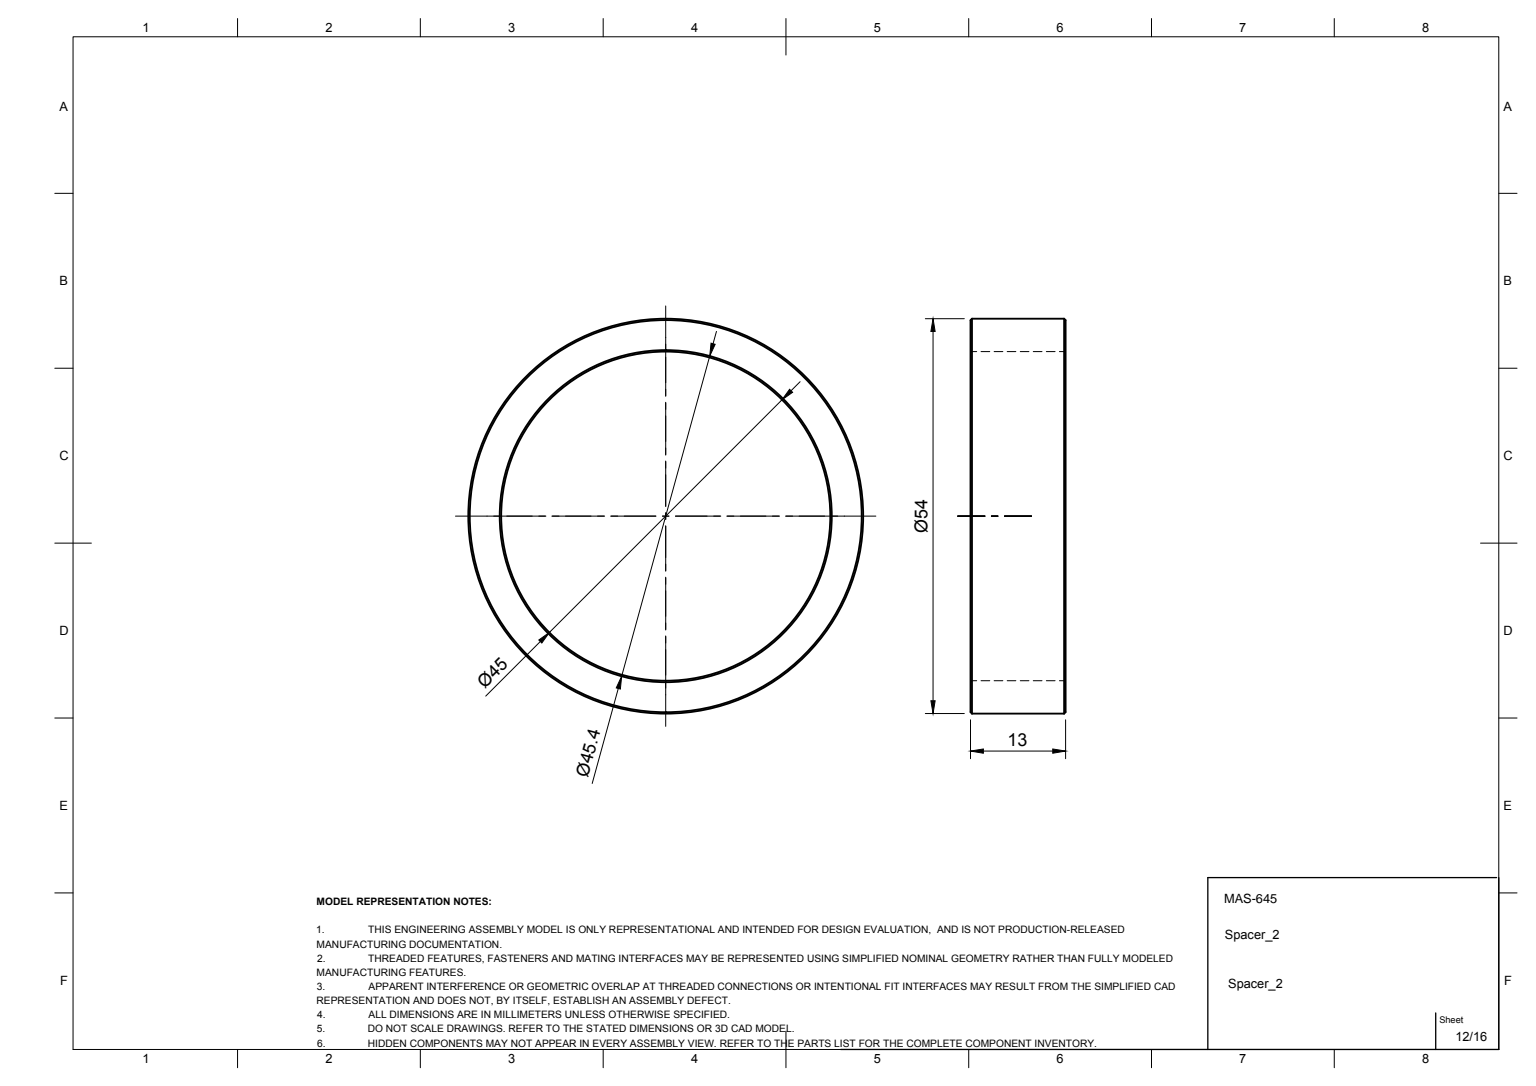
ISO-10303-21;
HEADER;
FILE_DESCRIPTION((''),'2;1');
FILE_NAME('Spacer_2.step','2026-10-09T10:54:55-07:00',(''),(''),'','','');
FILE_SCHEMA (('AUTOMOTIVE_DESIGN { 1 0 10303 214 3 1 1 }'));
ENDSEC;
DATA;
#10=MECHANICAL_DESIGN_GEOMETRIC_PRESENTATION_REPRESENTATION('',(#602),#63824);
#572=SHAPE_REPRESENTATION_RELATIONSHIP('SRR','None',#63886,#587) ;
#587=ADVANCED_BREP_SHAPE_REPRESENTATION('',(#617),#63816) ;
#602=STYLED_ITEM('',(#63963),#617) ;
#617=MANIFOLD_SOLID_BREP('Body1',#15501) ;
#748=FACE_BOUND('',#2811,.T.) ;
#749=FACE_BOUND('',#2817,.T.) ;
#906=PLANE('',#16195) ;
#907=PLANE('',#16205) ;
#1262=CYLINDRICAL_SURFACE('',#16197,27.) ;
#1263=CYLINDRICAL_SURFACE('',#16201,22.5) ;
#1825=FACE_OUTER_BOUND('',#2809,.T.) ;
#1826=FACE_OUTER_BOUND('',#2810,.T.) ;
#1827=FACE_OUTER_BOUND('',#2812,.T.) ;
#1828=FACE_OUTER_BOUND('',#2813,.T.) ;
#1829=FACE_OUTER_BOUND('',#2814,.T.) ;
#1830=FACE_OUTER_BOUND('',#2815,.T.) ;
#1831=FACE_OUTER_BOUND('',#2816,.T.) ;
#1832=FACE_OUTER_BOUND('',#2818,.T.) ;
#2809=EDGE_LOOP('',(#11030,#11031,#11032,#11033)) ;
#2810=EDGE_LOOP('',(#11034)) ;
#2811=EDGE_LOOP('',(#11035)) ;
#2812=EDGE_LOOP('',(#11036,#11037,#11038,#11039)) ;
#2813=EDGE_LOOP('',(#11040,#11041,#11042,#11043)) ;
#2814=EDGE_LOOP('',(#11044,#11045,#11046,#11047)) ;
#2815=EDGE_LOOP('',(#11048,#11049,#11050,#11051)) ;
#2816=EDGE_LOOP('',(#11052)) ;
#2817=EDGE_LOOP('',(#11053)) ;
#2818=EDGE_LOOP('',(#11054,#11055,#11056,#11057)) ;
#3701=CIRCLE('',#16193,27.) ;
#3702=CIRCLE('',#16194,26.8) ;
#3703=CIRCLE('',#16196,22.7) ;
#3704=CIRCLE('',#16198,27.) ;
#3705=CIRCLE('',#16200,22.5) ;
#3706=CIRCLE('',#16202,22.5) ;
#3707=CIRCLE('',#16204,26.8) ;
#3708=CIRCLE('',#16206,22.7) ;
#4958=LINE('',#51923,#5614) ;
#4959=LINE('',#51931,#5615) ;
#4960=LINE('',#51935,#5616) ;
#4961=LINE('',#51938,#5617) ;
#4962=LINE('',#51942,#5618) ;
#4963=LINE('',#51948,#5619) ;
#5614=VECTOR('',#19208,26.9) ;
#5615=VECTOR('',#19219,27.) ;
#5616=VECTOR('',#19224,22.6) ;
#5617=VECTOR('',#19227,22.5) ;
#5618=VECTOR('',#19232,26.9) ;
#5619=VECTOR('',#19241,22.6) ;
#6427=VERTEX_POINT('',#51920) ;
#6428=VERTEX_POINT('',#51922) ;
#6429=VERTEX_POINT('',#51926) ;
#6430=VERTEX_POINT('',#51929) ;
#6431=VERTEX_POINT('',#51933) ;
#6432=VERTEX_POINT('',#51937) ;
#6433=VERTEX_POINT('',#51941) ;
#6434=VERTEX_POINT('',#51945) ;
#8069=EDGE_CURVE('',#6427,#6427,#3701,.T.) ;
#8070=EDGE_CURVE('',#6427,#6428,#4958,.T.) ;
#8071=EDGE_CURVE('',#6428,#6428,#3702,.T.) ;
#8072=EDGE_CURVE('',#6429,#6429,#3703,.T.) ;
#8073=EDGE_CURVE('',#6430,#6430,#3704,.T.) ;
#8074=EDGE_CURVE('',#6430,#6427,#4959,.T.) ;
#8075=EDGE_CURVE('',#6431,#6431,#3705,.T.) ;
#8076=EDGE_CURVE('',#6431,#6429,#4960,.T.) ;
#8077=EDGE_CURVE('',#6431,#6432,#4961,.T.) ;
#8078=EDGE_CURVE('',#6432,#6432,#3706,.T.) ;
#8079=EDGE_CURVE('',#6430,#6433,#4962,.T.) ;
#8080=EDGE_CURVE('',#6433,#6433,#3707,.T.) ;
#8081=EDGE_CURVE('',#6434,#6434,#3708,.T.) ;
#8082=EDGE_CURVE('',#6432,#6434,#4963,.T.) ;
#11030=ORIENTED_EDGE('',*,*,#8069,.T.) ;
#11031=ORIENTED_EDGE('',*,*,#8070,.T.) ;
#11032=ORIENTED_EDGE('',*,*,#8071,.T.) ;
#11033=ORIENTED_EDGE('',*,*,#8070,.F.) ;
#11034=ORIENTED_EDGE('',*,*,#8071,.F.) ;
#11035=ORIENTED_EDGE('',*,*,#8072,.F.) ;
#11036=ORIENTED_EDGE('',*,*,#8073,.F.) ;
#11037=ORIENTED_EDGE('',*,*,#8074,.T.) ;
#11038=ORIENTED_EDGE('',*,*,#8069,.F.) ;
#11039=ORIENTED_EDGE('',*,*,#8074,.F.) ;
#11040=ORIENTED_EDGE('',*,*,#8075,.T.) ;
#11041=ORIENTED_EDGE('',*,*,#8076,.T.) ;
#11042=ORIENTED_EDGE('',*,*,#8072,.T.) ;
#11043=ORIENTED_EDGE('',*,*,#8076,.F.) ;
#11044=ORIENTED_EDGE('',*,*,#8075,.F.) ;
#11045=ORIENTED_EDGE('',*,*,#8077,.T.) ;
#11046=ORIENTED_EDGE('',*,*,#8078,.F.) ;
#11047=ORIENTED_EDGE('',*,*,#8077,.F.) ;
#11048=ORIENTED_EDGE('',*,*,#8073,.T.) ;
#11049=ORIENTED_EDGE('',*,*,#8079,.T.) ;
#11050=ORIENTED_EDGE('',*,*,#8080,.T.) ;
#11051=ORIENTED_EDGE('',*,*,#8079,.F.) ;
#11052=ORIENTED_EDGE('',*,*,#8080,.F.) ;
#11053=ORIENTED_EDGE('',*,*,#8081,.F.) ;
#11054=ORIENTED_EDGE('',*,*,#8078,.T.) ;
#11055=ORIENTED_EDGE('',*,*,#8082,.T.) ;
#11056=ORIENTED_EDGE('',*,*,#8081,.T.) ;
#11057=ORIENTED_EDGE('',*,*,#8082,.F.) ;
#14549=CONICAL_SURFACE('',#16192,26.9,0.785398163397449) ;
#14550=CONICAL_SURFACE('',#16199,22.6,0.785398163397449) ;
#14551=CONICAL_SURFACE('',#16203,26.9,0.785398163397448) ;
#14552=CONICAL_SURFACE('',#16207,22.6,0.785398163397448) ;
#14913=ADVANCED_FACE('',(#1825),#14549,.T.) ;
#14914=ADVANCED_FACE('',(#1826,#748),#906,.F.) ;
#14915=ADVANCED_FACE('',(#1827),#1262,.T.) ;
#14916=ADVANCED_FACE('',(#1828),#14550,.F.) ;
#14917=ADVANCED_FACE('',(#1829),#1263,.F.) ;
#14918=ADVANCED_FACE('',(#1830),#14551,.T.) ;
#14919=ADVANCED_FACE('',(#1831,#749),#907,.T.) ;
#14920=ADVANCED_FACE('',(#1832),#14552,.F.) ;
#15501=CLOSED_SHELL('',(#14913,#14914,#14915,#14916,#14917,#14918,#14919,
#14920)) ;
#16191=AXIS2_PLACEMENT_3D('',#51918,#19202,#19203) ;
#16192=AXIS2_PLACEMENT_3D('',#51919,#19204,#19205) ;
#16193=AXIS2_PLACEMENT_3D('',#51921,#19206,#19207) ;
#16194=AXIS2_PLACEMENT_3D('',#51924,#19209,#19210) ;
#16195=AXIS2_PLACEMENT_3D('',#51925,#19211,#19212) ;
#16196=AXIS2_PLACEMENT_3D('',#51927,#19213,#19214) ;
#16197=AXIS2_PLACEMENT_3D('',#51928,#19215,#19216) ;
#16198=AXIS2_PLACEMENT_3D('',#51930,#19217,#19218) ;
#16199=AXIS2_PLACEMENT_3D('',#51932,#19220,#19221) ;
#16200=AXIS2_PLACEMENT_3D('',#51934,#19222,#19223) ;
#16201=AXIS2_PLACEMENT_3D('',#51936,#19225,#19226) ;
#16202=AXIS2_PLACEMENT_3D('',#51939,#19228,#19229) ;
#16203=AXIS2_PLACEMENT_3D('',#51940,#19230,#19231) ;
#16204=AXIS2_PLACEMENT_3D('',#51943,#19233,#19234) ;
#16205=AXIS2_PLACEMENT_3D('',#51944,#19235,#19236) ;
#16206=AXIS2_PLACEMENT_3D('',#51946,#19237,#19238) ;
#16207=AXIS2_PLACEMENT_3D('',#51947,#19239,#19240) ;
#19202=DIRECTION('axis',(0.,0.,1.)) ;
#19203=DIRECTION('refdir',(1.,0.,0.)) ;
#19204=DIRECTION('center_axis',(0.,0.,1.)) ;
#19205=DIRECTION('ref_axis',(1.,0.,0.)) ;
#19206=DIRECTION('center_axis',(0.,0.,-1.)) ;
#19207=DIRECTION('ref_axis',(1.,0.,0.)) ;
#19208=DIRECTION('',(0.707106781186548,8.65956056235494E-17,-0.707106781186547)) ;
#19209=DIRECTION('center_axis',(0.,0.,1.)) ;
#19210=DIRECTION('ref_axis',(1.,0.,0.)) ;
#19211=DIRECTION('center_axis',(0.,0.,1.)) ;
#19212=DIRECTION('ref_axis',(1.,0.,0.)) ;
#19213=DIRECTION('center_axis',(0.,0.,-1.)) ;
#19214=DIRECTION('ref_axis',(1.,0.,0.)) ;
#19215=DIRECTION('center_axis',(0.,0.,1.)) ;
#19216=DIRECTION('ref_axis',(1.,0.,0.)) ;
#19217=DIRECTION('center_axis',(0.,0.,1.)) ;
#19218=DIRECTION('ref_axis',(1.,0.,0.)) ;
#19219=DIRECTION('',(0.,0.,-1.)) ;
#19220=DIRECTION('center_axis',(0.,0.,-1.)) ;
#19221=DIRECTION('ref_axis',(1.,0.,0.)) ;
#19222=DIRECTION('center_axis',(0.,0.,1.)) ;
#19223=DIRECTION('ref_axis',(1.,0.,0.)) ;
#19224=DIRECTION('',(-0.707106781186548,8.65956056235494E-17,-0.707106781186547)) ;
#19225=DIRECTION('center_axis',(0.,0.,1.)) ;
#19226=DIRECTION('ref_axis',(1.,0.,0.)) ;
#19227=DIRECTION('',(0.,0.,1.)) ;
#19228=DIRECTION('center_axis',(0.,0.,-1.)) ;
#19229=DIRECTION('ref_axis',(1.,0.,0.)) ;
#19230=DIRECTION('center_axis',(0.,0.,-1.)) ;
#19231=DIRECTION('ref_axis',(1.,0.,0.)) ;
#19232=DIRECTION('',(0.707106781186547,-8.65956056235493E-17,0.707106781186548)) ;
#19233=DIRECTION('center_axis',(0.,0.,-1.)) ;
#19234=DIRECTION('ref_axis',(1.,0.,0.)) ;
#19235=DIRECTION('center_axis',(0.,0.,1.)) ;
#19236=DIRECTION('ref_axis',(1.,0.,0.)) ;
#19237=DIRECTION('center_axis',(0.,0.,1.)) ;
#19238=DIRECTION('ref_axis',(1.,0.,0.)) ;
#19239=DIRECTION('center_axis',(0.,0.,1.)) ;
#19240=DIRECTION('ref_axis',(1.,0.,0.)) ;
#19241=DIRECTION('',(-0.707106781186547,-8.65956056235493E-17,0.707106781186548)) ;
#51918=CARTESIAN_POINT('',(0.,0.,0.)) ;
#51919=CARTESIAN_POINT('Origin',(0.,0.,0.1)) ;
#51920=CARTESIAN_POINT('',(-27.,3.30654635769785E-15,0.2)) ;
#51921=CARTESIAN_POINT('Origin',(0.,0.,0.2)) ;
#51922=CARTESIAN_POINT('',(-26.8,-3.28205342171491E-15,0.)) ;
#51923=CARTESIAN_POINT('',(-26.9,-3.29429988970638E-15,0.1)) ;
#51924=CARTESIAN_POINT('Origin',(0.,0.,0.)) ;
#51925=CARTESIAN_POINT('Origin',(0.,0.,0.)) ;
#51926=CARTESIAN_POINT('',(-22.7,2.77994823406449E-15,0.)) ;
#51927=CARTESIAN_POINT('Origin',(0.,0.,0.)) ;
#51928=CARTESIAN_POINT('Origin',(0.,0.,0.)) ;
#51929=CARTESIAN_POINT('',(-27.,-3.30654635769785E-15,12.8)) ;
#51930=CARTESIAN_POINT('Origin',(0.,0.,12.8)) ;
#51931=CARTESIAN_POINT('',(-27.,-3.30654635769785E-15,0.)) ;
#51932=CARTESIAN_POINT('Origin',(0.,0.,0.1)) ;
#51933=CARTESIAN_POINT('',(-22.5,-2.75545529808154E-15,0.2)) ;
#51934=CARTESIAN_POINT('Origin',(0.,0.,0.2)) ;
#51935=CARTESIAN_POINT('',(-22.6,2.76770176607302E-15,0.1)) ;
#51936=CARTESIAN_POINT('Origin',(0.,0.,0.)) ;
#51937=CARTESIAN_POINT('',(-22.5,2.75545529808154E-15,12.8)) ;
#51938=CARTESIAN_POINT('',(-22.5,-2.75545529808154E-15,0.)) ;
#51939=CARTESIAN_POINT('Origin',(0.,0.,12.8)) ;
#51940=CARTESIAN_POINT('Origin',(0.,0.,12.9)) ;
#51941=CARTESIAN_POINT('',(-26.8,3.28205342171491E-15,13.)) ;
#51942=CARTESIAN_POINT('',(-26.9,3.29429988970638E-15,12.9)) ;
#51943=CARTESIAN_POINT('Origin',(0.,0.,13.)) ;
#51944=CARTESIAN_POINT('Origin',(0.,0.,13.)) ;
#51945=CARTESIAN_POINT('',(-22.7,-2.77994823406449E-15,13.)) ;
#51946=CARTESIAN_POINT('Origin',(0.,0.,13.)) ;
#51947=CARTESIAN_POINT('Origin',(0.,0.,12.9)) ;
#51948=CARTESIAN_POINT('',(-22.6,-2.76770176607302E-15,12.9)) ;
#63799=UNCERTAINTY_MEASURE_WITH_UNIT(LENGTH_MEASURE(0.01),#63825,
'DISTANCE_ACCURACY_VALUE',
'Maximum model space distance between geometric entities at asserted c
onnectivities') ;
#63807=UNCERTAINTY_MEASURE_WITH_UNIT(LENGTH_MEASURE(0.01),#63825,
'DISTANCE_ACCURACY_VALUE',
'Maximum model space distance between geometric entities at asserted c
onnectivities') ;
#63816=(
GEOMETRIC_REPRESENTATION_CONTEXT(3)
GLOBAL_UNCERTAINTY_ASSIGNED_CONTEXT((#63799))
GLOBAL_UNIT_ASSIGNED_CONTEXT((#63825,#63827,#63828))
REPRESENTATION_CONTEXT('','3D')
) ;
#63824=(
GEOMETRIC_REPRESENTATION_CONTEXT(3)
GLOBAL_UNCERTAINTY_ASSIGNED_CONTEXT((#63807))
GLOBAL_UNIT_ASSIGNED_CONTEXT((#63825,#63827,#63828))
REPRESENTATION_CONTEXT('','3D')
) ;
#63825=(
LENGTH_UNIT()
NAMED_UNIT(*)
SI_UNIT(.MILLI.,.METRE.)
) ;
#63827=(
NAMED_UNIT(*)
PLANE_ANGLE_UNIT()
SI_UNIT($,.RADIAN.)
) ;
#63828=(
NAMED_UNIT(*)
SI_UNIT($,.STERADIAN.)
SOLID_ANGLE_UNIT()
) ;
#63837=SHAPE_DEFINITION_REPRESENTATION(#63853,#63886) ;
#63853=PRODUCT_DEFINITION_SHAPE('',$,#63903) ;
#63886=SHAPE_REPRESENTATION('',(#16191),#63816) ;
#63894=PRODUCT_DEFINITION_CONTEXT('part definition',#63944,'design') ;
#63903=PRODUCT_DEFINITION('Spacer_2','Spacer_2',#63919,#63894) ;
#63919=PRODUCT_DEFINITION_FORMATION('',$,#63954) ;
#63944=APPLICATION_CONTEXT(
'Core Data for Automotive Mechanical Design Process') ;
#63945=PRODUCT_CONTEXT('part definition',#63944,'mechanical') ;
#63954=PRODUCT('Spacer_2','Spacer_2',$,(#63945)) ;
#63963=PRESENTATION_STYLE_ASSIGNMENT((#63968)) ;
#63968=SURFACE_STYLE_USAGE(.BOTH.,#63973) ;
#63973=SURFACE_SIDE_STYLE('',(#63978)) ;
#63978=SURFACE_STYLE_FILL_AREA(#63983) ;
#63983=FILL_AREA_STYLE('Opaque(160,160,160)',(#63988)) ;
#63988=FILL_AREA_STYLE_COLOUR('Opaque(160,160,160)',#63993) ;
#63993=COLOUR_RGB('Opaque(160,160,160)', 0.09019608, 0.27058824, 0.51372549) ;
ENDSEC;
END-ISO-10303-21;
